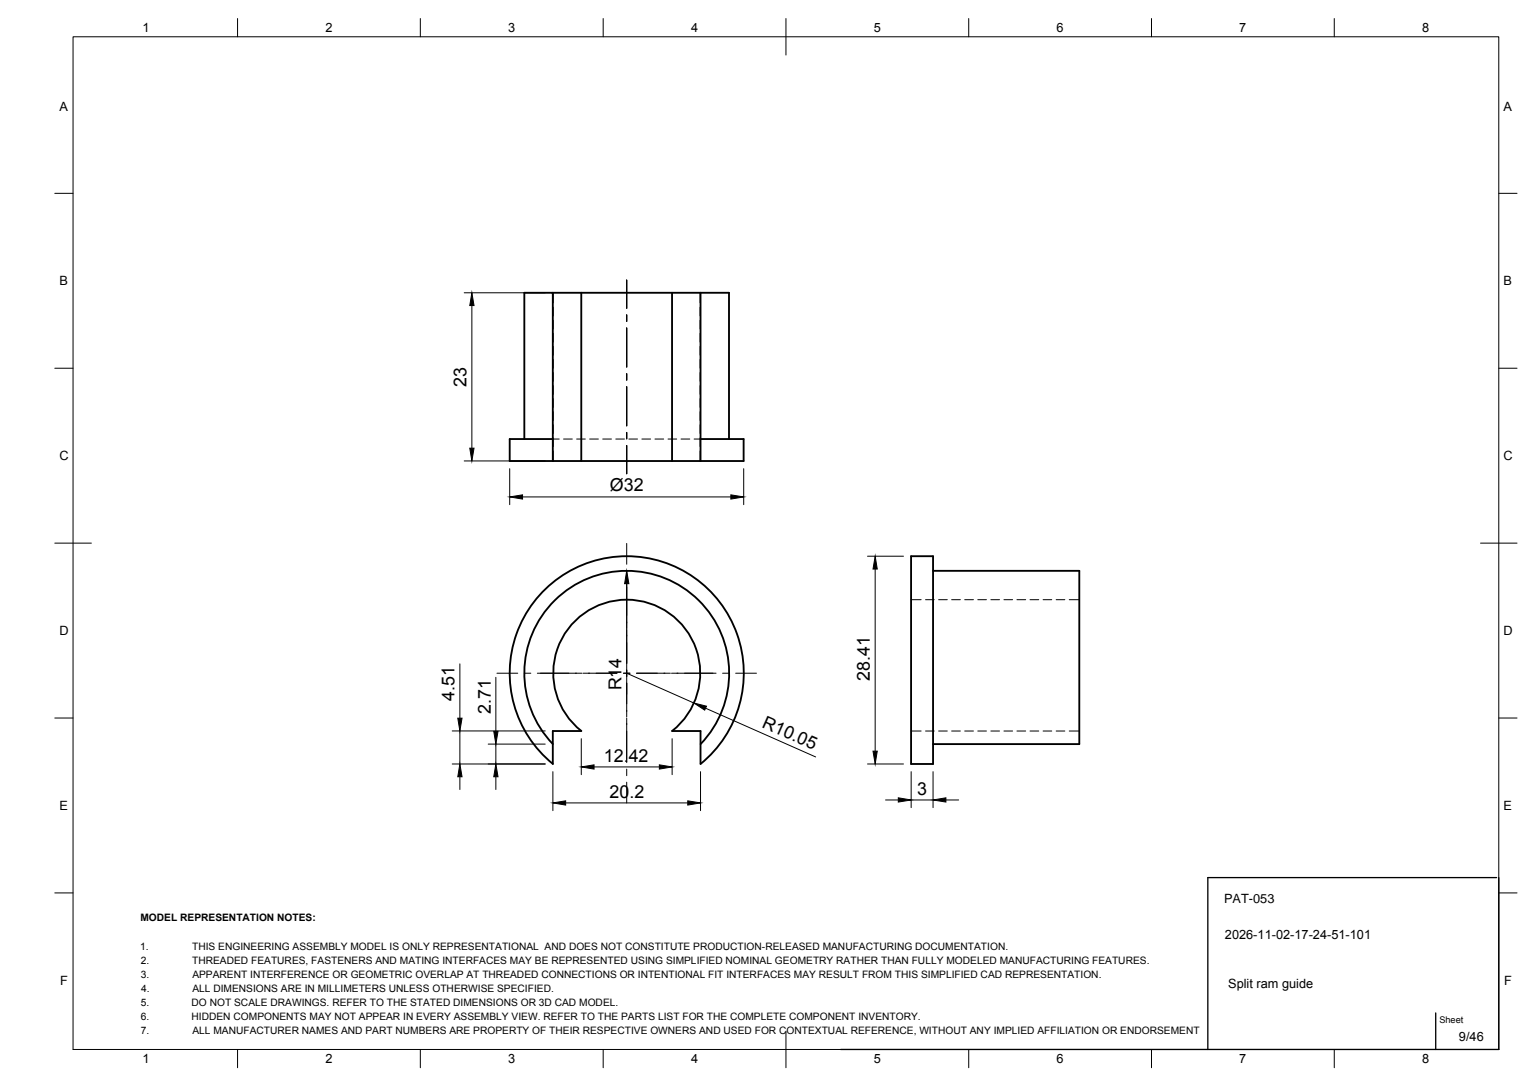
ISO-10303-21;
HEADER;
/* Generated by software containing ST-Developer
 * from STEP Tools, Inc. (www.steptools.com) 
 */

FILE_DESCRIPTION(
/* description */ ('Hand-operated arbor press'),
/* implementation_level */ '2;1');

FILE_NAME(
/* name */ 'Split ram guide.step',
/* time_stamp */ '2026-10-28T03:25:25-07:00',
/* author */ (''),
/* organization */ (''),
/* preprocessor_version */ 'ST-DEVELOPER v20.2',
/* originating_system */ 'Autodesk Translation Framework v15.17.0.0',
/* authorisation */ '');

FILE_SCHEMA (('AUTOMOTIVE_DESIGN { 1 0 10303 214 3 1 1 }'));
ENDSEC;

DATA;
#10=MECHANICAL_DESIGN_GEOMETRIC_PRESENTATION_REPRESENTATION('',(#590),#32751);
#506=SHAPE_REPRESENTATION_RELATIONSHIP('SRR','None',#32935,#548);
#548=ADVANCED_BREP_SHAPE_REPRESENTATION('',(#639),#32709);
#590=STYLED_ITEM('',(#33235),#639);
#639=MANIFOLD_SOLID_BREP('Body1',#12487);
#894=PLANE('',#13123);
#895=PLANE('',#13124);
#896=PLANE('',#13125);
#897=PLANE('',#13126);
#898=PLANE('',#13127);
#899=PLANE('',#13134);
#900=PLANE('',#13138);
#1362=FACE_OUTER_BOUND('',#2078,.T.);
#1363=FACE_OUTER_BOUND('',#2079,.T.);
#1364=FACE_OUTER_BOUND('',#2080,.T.);
#1365=FACE_OUTER_BOUND('',#2081,.T.);
#1366=FACE_OUTER_BOUND('',#2082,.T.);
#1367=FACE_OUTER_BOUND('',#2083,.T.);
#1368=FACE_OUTER_BOUND('',#2084,.T.);
#1369=FACE_OUTER_BOUND('',#2085,.T.);
#1370=FACE_OUTER_BOUND('',#2086,.T.);
#1371=FACE_OUTER_BOUND('',#2087,.T.);
#2078=EDGE_LOOP('',(#8648,#8649,#8650,#8651));
#2079=EDGE_LOOP('',(#8652,#8653,#8654,#8655));
#2080=EDGE_LOOP('',(#8656,#8657,#8658,#8659,#8660,#8661));
#2081=EDGE_LOOP('',(#8662,#8663,#8664,#8665,#8666,#8667));
#2082=EDGE_LOOP('',(#8668,#8669,#8670,#8671,#8672,#8673));
#2083=EDGE_LOOP('',(#8674,#8675,#8676,#8677));
#2084=EDGE_LOOP('',(#8678,#8679,#8680,#8681));
#2085=EDGE_LOOP('',(#8682,#8683,#8684,#8685));
#2086=EDGE_LOOP('',(#8686,#8687,#8688,#8689));
#2087=EDGE_LOOP('',(#8690,#8691,#8692,#8693,#8694,#8695));
#2938=LINE('',#17987,#4109);
#2939=LINE('',#17989,#4110);
#2940=LINE('',#17991,#4111);
#2941=LINE('',#17992,#4112);
#2942=LINE('',#17996,#4113);
#2943=LINE('',#17998,#4114);
#2944=LINE('',#18000,#4115);
#2945=LINE('',#18001,#4116);
#2946=LINE('',#18004,#4117);
#2947=LINE('',#18006,#4118);
#2948=LINE('',#18008,#4119);
#2949=LINE('',#18010,#4120);
#2950=LINE('',#18011,#4121);
#2951=LINE('',#18014,#4122);
#2952=LINE('',#18016,#4123);
#2953=LINE('',#18018,#4124);
#2954=LINE('',#18020,#4125);
#2955=LINE('',#18021,#4126);
#4109=VECTOR('',#14519,1.);
#4110=VECTOR('',#14520,1.);
#4111=VECTOR('',#14521,1.);
#4112=VECTOR('',#14522,1.);
#4113=VECTOR('',#14525,1.);
#4114=VECTOR('',#14526,1.);
#4115=VECTOR('',#14527,1.);
#4116=VECTOR('',#14528,1.);
#4117=VECTOR('',#14531,1.);
#4118=VECTOR('',#14532,1.);
#4119=VECTOR('',#14533,1.);
#4120=VECTOR('',#14534,1.);
#4121=VECTOR('',#14535,1.);
#4122=VECTOR('',#14538,1.);
#4123=VECTOR('',#14539,1.);
#4124=VECTOR('',#14540,1.);
#4125=VECTOR('',#14541,1.);
#4126=VECTOR('',#14542,1.);
#5214=CIRCLE('',#13128,1.4);
#5215=CIRCLE('',#13129,1.005);
#5216=CIRCLE('',#13131,1.005);
#5217=CIRCLE('',#13133,1.4);
#5218=CIRCLE('',#13135,1.6);
#5219=CIRCLE('',#13137,1.6);
#5664=VERTEX_POINT('',#17985);
#5665=VERTEX_POINT('',#17986);
#5666=VERTEX_POINT('',#17988);
#5667=VERTEX_POINT('',#17990);
#5668=VERTEX_POINT('',#17994);
#5669=VERTEX_POINT('',#17995);
#5670=VERTEX_POINT('',#17997);
#5671=VERTEX_POINT('',#17999);
#5672=VERTEX_POINT('',#18003);
#5673=VERTEX_POINT('',#18005);
#5674=VERTEX_POINT('',#18007);
#5675=VERTEX_POINT('',#18009);
#5676=VERTEX_POINT('',#18013);
#5677=VERTEX_POINT('',#18015);
#5678=VERTEX_POINT('',#18017);
#5679=VERTEX_POINT('',#18019);
#6827=EDGE_CURVE('',#5664,#5665,#2938,.T.);
#6828=EDGE_CURVE('',#5664,#5666,#2939,.T.);
#6829=EDGE_CURVE('',#5667,#5666,#2940,.T.);
#6830=EDGE_CURVE('',#5665,#5667,#2941,.T.);
#6831=EDGE_CURVE('',#5668,#5669,#2942,.T.);
#6832=EDGE_CURVE('',#5670,#5668,#2943,.T.);
#6833=EDGE_CURVE('',#5671,#5670,#2944,.T.);
#6834=EDGE_CURVE('',#5669,#5671,#2945,.T.);
#6835=EDGE_CURVE('',#5672,#5668,#2946,.T.);
#6836=EDGE_CURVE('',#5673,#5672,#2947,.T.);
#6837=EDGE_CURVE('',#5674,#5673,#2948,.T.);
#6838=EDGE_CURVE('',#5675,#5674,#2949,.T.);
#6839=EDGE_CURVE('',#5670,#5675,#2950,.T.);
#6840=EDGE_CURVE('',#5676,#5664,#2951,.T.);
#6841=EDGE_CURVE('',#5677,#5676,#2952,.T.);
#6842=EDGE_CURVE('',#5678,#5677,#2953,.T.);
#6843=EDGE_CURVE('',#5679,#5678,#2954,.T.);
#6844=EDGE_CURVE('',#5666,#5679,#2955,.T.);
#6845=EDGE_CURVE('',#5676,#5675,#5214,.T.);
#6846=EDGE_CURVE('',#5671,#5665,#5215,.T.);
#6847=EDGE_CURVE('',#5669,#5667,#5216,.T.);
#6848=EDGE_CURVE('',#5677,#5674,#5217,.T.);
#6849=EDGE_CURVE('',#5678,#5673,#5218,.T.);
#6850=EDGE_CURVE('',#5679,#5672,#5219,.T.);
#8648=ORIENTED_EDGE('',*,*,#6827,.F.);
#8649=ORIENTED_EDGE('',*,*,#6828,.T.);
#8650=ORIENTED_EDGE('',*,*,#6829,.F.);
#8651=ORIENTED_EDGE('',*,*,#6830,.F.);
#8652=ORIENTED_EDGE('',*,*,#6831,.F.);
#8653=ORIENTED_EDGE('',*,*,#6832,.F.);
#8654=ORIENTED_EDGE('',*,*,#6833,.F.);
#8655=ORIENTED_EDGE('',*,*,#6834,.F.);
#8656=ORIENTED_EDGE('',*,*,#6835,.F.);
#8657=ORIENTED_EDGE('',*,*,#6836,.F.);
#8658=ORIENTED_EDGE('',*,*,#6837,.F.);
#8659=ORIENTED_EDGE('',*,*,#6838,.F.);
#8660=ORIENTED_EDGE('',*,*,#6839,.F.);
#8661=ORIENTED_EDGE('',*,*,#6832,.T.);
#8662=ORIENTED_EDGE('',*,*,#6840,.F.);
#8663=ORIENTED_EDGE('',*,*,#6841,.F.);
#8664=ORIENTED_EDGE('',*,*,#6842,.F.);
#8665=ORIENTED_EDGE('',*,*,#6843,.F.);
#8666=ORIENTED_EDGE('',*,*,#6844,.F.);
#8667=ORIENTED_EDGE('',*,*,#6828,.F.);
#8668=ORIENTED_EDGE('',*,*,#6833,.T.);
#8669=ORIENTED_EDGE('',*,*,#6839,.T.);
#8670=ORIENTED_EDGE('',*,*,#6845,.F.);
#8671=ORIENTED_EDGE('',*,*,#6840,.T.);
#8672=ORIENTED_EDGE('',*,*,#6827,.T.);
#8673=ORIENTED_EDGE('',*,*,#6846,.F.);
#8674=ORIENTED_EDGE('',*,*,#6834,.T.);
#8675=ORIENTED_EDGE('',*,*,#6846,.T.);
#8676=ORIENTED_EDGE('',*,*,#6830,.T.);
#8677=ORIENTED_EDGE('',*,*,#6847,.F.);
#8678=ORIENTED_EDGE('',*,*,#6838,.T.);
#8679=ORIENTED_EDGE('',*,*,#6848,.F.);
#8680=ORIENTED_EDGE('',*,*,#6841,.T.);
#8681=ORIENTED_EDGE('',*,*,#6845,.T.);
#8682=ORIENTED_EDGE('',*,*,#6837,.T.);
#8683=ORIENTED_EDGE('',*,*,#6849,.F.);
#8684=ORIENTED_EDGE('',*,*,#6842,.T.);
#8685=ORIENTED_EDGE('',*,*,#6848,.T.);
#8686=ORIENTED_EDGE('',*,*,#6836,.T.);
#8687=ORIENTED_EDGE('',*,*,#6850,.F.);
#8688=ORIENTED_EDGE('',*,*,#6843,.T.);
#8689=ORIENTED_EDGE('',*,*,#6849,.T.);
#8690=ORIENTED_EDGE('',*,*,#6831,.T.);
#8691=ORIENTED_EDGE('',*,*,#6847,.T.);
#8692=ORIENTED_EDGE('',*,*,#6829,.T.);
#8693=ORIENTED_EDGE('',*,*,#6844,.T.);
#8694=ORIENTED_EDGE('',*,*,#6850,.T.);
#8695=ORIENTED_EDGE('',*,*,#6835,.T.);
#11666=CYLINDRICAL_SURFACE('',#13130,1.005);
#11667=CYLINDRICAL_SURFACE('',#13132,1.4);
#11668=CYLINDRICAL_SURFACE('',#13136,1.6);
#11871=ADVANCED_FACE('',(#1362),#894,.F.);
#11872=ADVANCED_FACE('',(#1363),#895,.F.);
#11873=ADVANCED_FACE('',(#1364),#896,.F.);
#11874=ADVANCED_FACE('',(#1365),#897,.F.);
#11875=ADVANCED_FACE('',(#1366),#898,.F.);
#11876=ADVANCED_FACE('',(#1367),#11666,.F.);
#11877=ADVANCED_FACE('',(#1368),#11667,.T.);
#11878=ADVANCED_FACE('',(#1369),#899,.F.);
#11879=ADVANCED_FACE('',(#1370),#11668,.T.);
#11880=ADVANCED_FACE('',(#1371),#900,.T.);
#12487=CLOSED_SHELL('',(#11871,#11872,#11873,#11874,#11875,#11876,#11877,
#11878,#11879,#11880));
#13122=AXIS2_PLACEMENT_3D('',#17983,#14515,#14516);
#13123=AXIS2_PLACEMENT_3D('',#17984,#14517,#14518);
#13124=AXIS2_PLACEMENT_3D('',#17993,#14523,#14524);
#13125=AXIS2_PLACEMENT_3D('',#18002,#14529,#14530);
#13126=AXIS2_PLACEMENT_3D('',#18012,#14536,#14537);
#13127=AXIS2_PLACEMENT_3D('',#18022,#14543,#14544);
#13128=AXIS2_PLACEMENT_3D('',#18023,#14545,#14546);
#13129=AXIS2_PLACEMENT_3D('',#18024,#14547,#14548);
#13130=AXIS2_PLACEMENT_3D('',#18025,#14549,#14550);
#13131=AXIS2_PLACEMENT_3D('',#18026,#14551,#14552);
#13132=AXIS2_PLACEMENT_3D('',#18027,#14553,#14554);
#13133=AXIS2_PLACEMENT_3D('',#18028,#14555,#14556);
#13134=AXIS2_PLACEMENT_3D('',#18029,#14557,#14558);
#13135=AXIS2_PLACEMENT_3D('',#18030,#14559,#14560);
#13136=AXIS2_PLACEMENT_3D('',#18031,#14561,#14562);
#13137=AXIS2_PLACEMENT_3D('',#18032,#14563,#14564);
#13138=AXIS2_PLACEMENT_3D('',#18033,#14565,#14566);
#14515=DIRECTION('axis',(0.,0.,1.));
#14516=DIRECTION('refdir',(1.,0.,0.));
#14517=DIRECTION('center_axis',(1.,0.,0.));
#14518=DIRECTION('ref_axis',(0.,1.,0.));
#14519=DIRECTION('',(0.,1.,0.));
#14520=DIRECTION('',(0.,0.,1.));
#14521=DIRECTION('',(0.,-1.,0.));
#14522=DIRECTION('',(0.,0.,1.));
#14523=DIRECTION('center_axis',(1.,0.,0.));
#14524=DIRECTION('ref_axis',(0.,1.,0.));
#14525=DIRECTION('',(0.,-1.,0.));
#14526=DIRECTION('',(0.,0.,1.));
#14527=DIRECTION('',(0.,1.,0.));
#14528=DIRECTION('',(0.,0.,-1.));
#14529=DIRECTION('center_axis',(0.,1.,0.));
#14530=DIRECTION('ref_axis',(-1.,0.,0.));
#14531=DIRECTION('',(1.,0.,0.));
#14532=DIRECTION('',(0.,0.,1.));
#14533=DIRECTION('',(-1.,0.,0.));
#14534=DIRECTION('',(0.,0.,1.));
#14535=DIRECTION('',(-1.,0.,0.));
#14536=DIRECTION('center_axis',(0.,-1.,0.));
#14537=DIRECTION('ref_axis',(1.,0.,0.));
#14538=DIRECTION('',(1.,0.,0.));
#14539=DIRECTION('',(0.,0.,-1.));
#14540=DIRECTION('',(1.,0.,0.));
#14541=DIRECTION('',(0.,0.,-1.));
#14542=DIRECTION('',(-1.,0.,0.));
#14543=DIRECTION('center_axis',(0.,0.,1.));
#14544=DIRECTION('ref_axis',(1.,0.,0.));
#14545=DIRECTION('center_axis',(0.,0.,1.));
#14546=DIRECTION('ref_axis',(1.,0.,0.));
#14547=DIRECTION('center_axis',(0.,0.,-1.));
#14548=DIRECTION('ref_axis',(1.,0.,0.));
#14549=DIRECTION('center_axis',(0.,0.,1.));
#14550=DIRECTION('ref_axis',(1.,0.,0.));
#14551=DIRECTION('center_axis',(0.,0.,-1.));
#14552=DIRECTION('ref_axis',(1.,0.,0.));
#14553=DIRECTION('center_axis',(0.,0.,1.));
#14554=DIRECTION('ref_axis',(1.,0.,0.));
#14555=DIRECTION('center_axis',(0.,0.,1.));
#14556=DIRECTION('ref_axis',(1.,0.,0.));
#14557=DIRECTION('center_axis',(0.,0.,1.));
#14558=DIRECTION('ref_axis',(1.,0.,0.));
#14559=DIRECTION('center_axis',(0.,0.,1.));
#14560=DIRECTION('ref_axis',(1.,0.,0.));
#14561=DIRECTION('center_axis',(0.,0.,1.));
#14562=DIRECTION('ref_axis',(1.,0.,0.));
#14563=DIRECTION('center_axis',(0.,0.,1.));
#14564=DIRECTION('ref_axis',(1.,0.,0.));
#14565=DIRECTION('center_axis',(0.,0.,1.));
#14566=DIRECTION('ref_axis',(1.,0.,0.));
#17983=CARTESIAN_POINT('',(0.,0.,0.));
#17984=CARTESIAN_POINT('Origin',(0.21,-1.01,12.9));
#17985=CARTESIAN_POINT('',(0.21,-1.01,13.));
#17986=CARTESIAN_POINT('',(0.21,-0.621228621362538,13.));
#17987=CARTESIAN_POINT('',(0.21,-0.505,13.));
#17988=CARTESIAN_POINT('',(0.21,-1.01,15.3));
#17989=CARTESIAN_POINT('',(0.21,-1.01,12.9));
#17990=CARTESIAN_POINT('',(0.21,-0.621228621362538,15.3));
#17991=CARTESIAN_POINT('',(0.21,-0.505,15.3));
#17992=CARTESIAN_POINT('',(0.21,-0.621228621362538,13.));
#17993=CARTESIAN_POINT('Origin',(0.21,-1.01,12.9));
#17994=CARTESIAN_POINT('',(0.21,1.01,15.3));
#17995=CARTESIAN_POINT('',(0.21,0.621228621362538,15.3));
#17996=CARTESIAN_POINT('',(0.21,-0.505,15.3));
#17997=CARTESIAN_POINT('',(0.21,1.01,13.));
#17998=CARTESIAN_POINT('',(0.21,1.01,12.9));
#17999=CARTESIAN_POINT('',(0.21,0.621228621362538,13.));
#18000=CARTESIAN_POINT('',(0.21,-0.505,13.));
#18001=CARTESIAN_POINT('',(0.21,0.621228621362538,13.));
#18002=CARTESIAN_POINT('Origin',(0.21,1.01,12.9));
#18003=CARTESIAN_POINT('',(-0.240927072796786,1.01,15.3));
#18004=CARTESIAN_POINT('',(0.605,1.01,15.3));
#18005=CARTESIAN_POINT('',(-0.240927072796786,1.01,15.));
#18006=CARTESIAN_POINT('',(-0.240927072796786,1.01,15.));
#18007=CARTESIAN_POINT('',(0.0305156009506911,1.01,15.));
#18008=CARTESIAN_POINT('',(0.605,1.01,15.));
#18009=CARTESIAN_POINT('',(0.0305156009506911,1.01,13.));
#18010=CARTESIAN_POINT('',(0.0305156009506911,1.01,13.));
#18011=CARTESIAN_POINT('',(0.605,1.01,13.));
#18012=CARTESIAN_POINT('Origin',(-0.7,-1.01,12.9));
#18013=CARTESIAN_POINT('',(0.0305156009506911,-1.01,13.));
#18014=CARTESIAN_POINT('',(0.15,-1.01,13.));
#18015=CARTESIAN_POINT('',(0.0305156009506911,-1.01,15.));
#18016=CARTESIAN_POINT('',(0.0305156009506911,-1.01,13.));
#18017=CARTESIAN_POINT('',(-0.240927072796786,-1.01,15.));
#18018=CARTESIAN_POINT('',(0.15,-1.01,15.));
#18019=CARTESIAN_POINT('',(-0.240927072796786,-1.01,15.3));
#18020=CARTESIAN_POINT('',(-0.240927072796786,-1.01,15.));
#18021=CARTESIAN_POINT('',(0.15,-1.01,15.3));
#18022=CARTESIAN_POINT('Origin',(1.,0.,13.));
#18023=CARTESIAN_POINT('Origin',(1.,0.,13.));
#18024=CARTESIAN_POINT('Origin',(1.,0.,13.));
#18025=CARTESIAN_POINT('Origin',(1.,0.,13.));
#18026=CARTESIAN_POINT('Origin',(1.,0.,15.3));
#18027=CARTESIAN_POINT('Origin',(1.,0.,13.));
#18028=CARTESIAN_POINT('Origin',(1.,0.,15.));
#18029=CARTESIAN_POINT('Origin',(1.,0.,15.));
#18030=CARTESIAN_POINT('Origin',(1.,0.,15.));
#18031=CARTESIAN_POINT('Origin',(1.,0.,15.));
#18032=CARTESIAN_POINT('Origin',(1.,0.,15.3));
#18033=CARTESIAN_POINT('Origin',(1.,0.,15.3));
#32660=UNCERTAINTY_MEASURE_WITH_UNIT(LENGTH_MEASURE(0.001),#32752,
'DISTANCE_ACCURACY_VALUE',
'Maximum model space distance between geometric entities at asserted c
onnectivities');
#32702=UNCERTAINTY_MEASURE_WITH_UNIT(LENGTH_MEASURE(0.001),#32752,
'DISTANCE_ACCURACY_VALUE',
'Maximum model space distance between geometric entities at asserted c
onnectivities');
#32709=(
GEOMETRIC_REPRESENTATION_CONTEXT(3)
GLOBAL_UNCERTAINTY_ASSIGNED_CONTEXT((#32660))
GLOBAL_UNIT_ASSIGNED_CONTEXT((#32752,#32754,#32755))
REPRESENTATION_CONTEXT('','3D')
);
#32751=(
GEOMETRIC_REPRESENTATION_CONTEXT(3)
GLOBAL_UNCERTAINTY_ASSIGNED_CONTEXT((#32702))
GLOBAL_UNIT_ASSIGNED_CONTEXT((#32752,#32754,#32755))
REPRESENTATION_CONTEXT('','3D')
);
#32752=(
LENGTH_UNIT()
NAMED_UNIT(*)
SI_UNIT(.CENTI.,.METRE.)
);
#32754=(
NAMED_UNIT(*)
PLANE_ANGLE_UNIT()
SI_UNIT($,.RADIAN.)
);
#32755=(
NAMED_UNIT(*)
SI_UNIT($,.STERADIAN.)
SOLID_ANGLE_UNIT()
);
#32762=SHAPE_DEFINITION_REPRESENTATION(#32810,#32935);
#32810=PRODUCT_DEFINITION_SHAPE('',$,#32984);
#32935=SHAPE_REPRESENTATION('',(#13122),#32709);
#32977=PRODUCT_DEFINITION_CONTEXT('part definition',#33123,'design');
#32984=PRODUCT_DEFINITION('Split ram guide','Split ram guide',#33032,#32977);
#33032=PRODUCT_DEFINITION_FORMATION('',$,#33131);
#33123=APPLICATION_CONTEXT(
'Core Data for Automotive Mechanical Design Process');
#33124=PRODUCT_CONTEXT('part definition',#33123,'mechanical');
#33131=PRODUCT('Split ram guide','Split ram guide','Split ram guide',(#33124));
#33229=COLOUR_RGB('Sky Blue',0.24,0.69,0.87);
#33230=FILL_AREA_STYLE_COLOUR('',#33229);
#33231=FILL_AREA_STYLE('',(#33230));
#33232=SURFACE_STYLE_FILL_AREA(#33231);
#33233=SURFACE_SIDE_STYLE('',(#33232));
#33234=SURFACE_STYLE_USAGE(.BOTH.,#33233);
#33235=PRESENTATION_STYLE_ASSIGNMENT((#33234));
ENDSEC;
END-ISO-10303-21;
